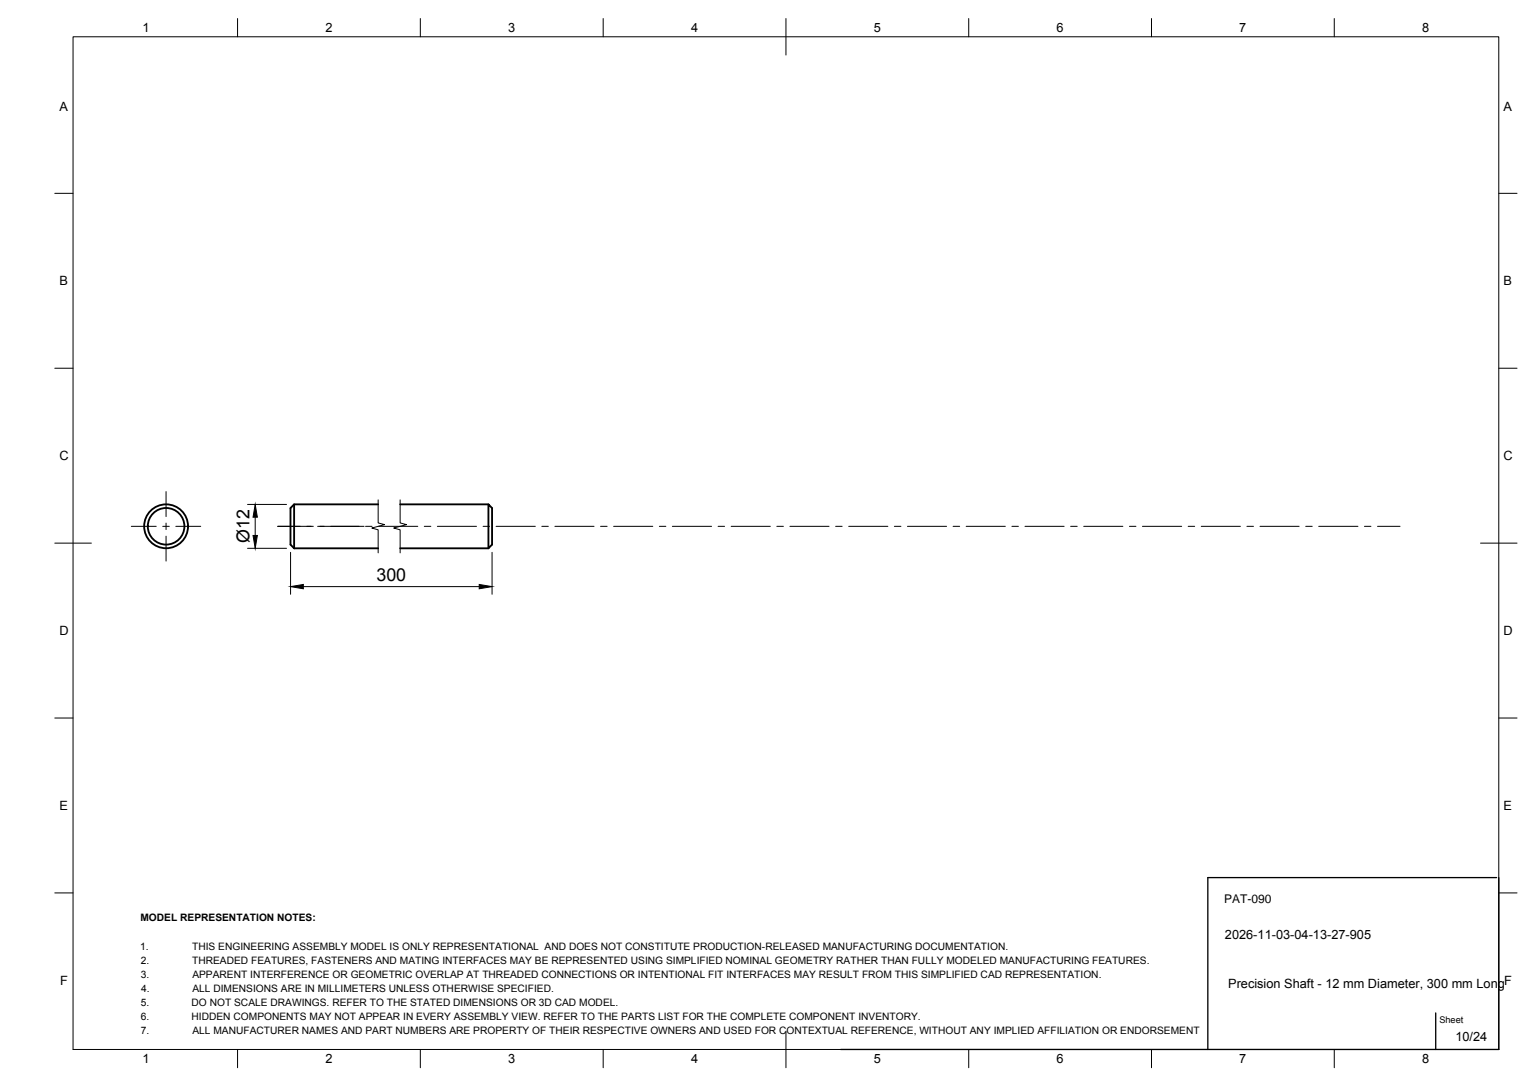
ISO-10303-21;
HEADER;
/* Generated by software containing ST-Developer
 * from STEP Tools, Inc. (www.steptools.com) 
 */

FILE_DESCRIPTION(
/* description */ ('Round-Shaft Linear Stage with Ball Bushings'),
/* implementation_level */ '2;1');

FILE_NAME(
/* name */ 'Precision Shaft - 12 mm Diameter, 300 mm Long.step',
/* time_stamp */ '2026-10-27T10:47:55-07:00',
/* author */ (''),
/* organization */ (''),
/* preprocessor_version */ 'ST-DEVELOPER v20.2',
/* originating_system */ 'Autodesk Translation Framework v15.17.0.0',
/* authorisation */ '');

FILE_SCHEMA (('AUTOMOTIVE_DESIGN { 1 0 10303 214 3 1 1 }'));
ENDSEC;

DATA;
#10=MECHANICAL_DESIGN_GEOMETRIC_PRESENTATION_REPRESENTATION('',(#307),#7835);
#243=CONICAL_SURFACE('',#4751,0.55,0.785398163397448);
#244=CONICAL_SURFACE('',#4757,0.55,0.785398163397441);
#265=SHAPE_REPRESENTATION_RELATIONSHIP('SRR','None',#7953,#286);
#286=ADVANCED_BREP_SHAPE_REPRESENTATION('',(#328),#7817);
#307=STYLED_ITEM('',(#8144),#328);
#328=MANIFOLD_SOLID_BREP('Body1',#4397);
#493=PLANE('',#4756);
#494=PLANE('',#4759);
#670=FACE_OUTER_BOUND('',#963,.T.);
#671=FACE_OUTER_BOUND('',#964,.T.);
#672=FACE_OUTER_BOUND('',#965,.T.);
#673=FACE_OUTER_BOUND('',#966,.T.);
#674=FACE_OUTER_BOUND('',#967,.T.);
#963=EDGE_LOOP('',(#3234,#3235,#3236,#3237));
#964=EDGE_LOOP('',(#3238,#3239,#3240,#3241));
#965=EDGE_LOOP('',(#3242));
#966=EDGE_LOOP('',(#3243,#3244,#3245,#3246));
#967=EDGE_LOOP('',(#3247));
#1329=LINE('',#6836,#1669);
#1330=LINE('',#6841,#1670);
#1331=LINE('',#6846,#1671);
#1669=VECTOR('',#5464,0.55);
#1670=VECTOR('',#5471,0.6);
#1671=VECTOR('',#5478,0.55);
#1969=CIRCLE('',#4752,0.6);
#1970=CIRCLE('',#4753,0.5);
#1971=CIRCLE('',#4755,0.6);
#1972=CIRCLE('',#4758,0.5);
#2198=VERTEX_POINT('',#6833);
#2199=VERTEX_POINT('',#6835);
#2200=VERTEX_POINT('',#6839);
#2201=VERTEX_POINT('',#6844);
#2585=EDGE_CURVE('',#2198,#2198,#1969,.T.);
#2586=EDGE_CURVE('',#2198,#2199,#1329,.T.);
#2587=EDGE_CURVE('',#2199,#2199,#1970,.T.);
#2588=EDGE_CURVE('',#2200,#2200,#1971,.T.);
#2589=EDGE_CURVE('',#2200,#2198,#1330,.T.);
#2590=EDGE_CURVE('',#2201,#2201,#1972,.T.);
#2591=EDGE_CURVE('',#2201,#2200,#1331,.T.);
#3234=ORIENTED_EDGE('',*,*,#2585,.T.);
#3235=ORIENTED_EDGE('',*,*,#2586,.T.);
#3236=ORIENTED_EDGE('',*,*,#2587,.T.);
#3237=ORIENTED_EDGE('',*,*,#2586,.F.);
#3238=ORIENTED_EDGE('',*,*,#2588,.F.);
#3239=ORIENTED_EDGE('',*,*,#2589,.T.);
#3240=ORIENTED_EDGE('',*,*,#2585,.F.);
#3241=ORIENTED_EDGE('',*,*,#2589,.F.);
#3242=ORIENTED_EDGE('',*,*,#2587,.F.);
#3243=ORIENTED_EDGE('',*,*,#2590,.T.);
#3244=ORIENTED_EDGE('',*,*,#2591,.T.);
#3245=ORIENTED_EDGE('',*,*,#2588,.T.);
#3246=ORIENTED_EDGE('',*,*,#2591,.F.);
#3247=ORIENTED_EDGE('',*,*,#2590,.F.);
#4072=CYLINDRICAL_SURFACE('',#4754,0.6);
#4189=ADVANCED_FACE('',(#670),#243,.T.);
#4190=ADVANCED_FACE('',(#671),#4072,.T.);
#4191=ADVANCED_FACE('',(#672),#493,.F.);
#4192=ADVANCED_FACE('',(#673),#244,.T.);
#4193=ADVANCED_FACE('',(#674),#494,.T.);
#4397=CLOSED_SHELL('',(#4189,#4190,#4191,#4192,#4193));
#4750=AXIS2_PLACEMENT_3D('',#6831,#5458,#5459);
#4751=AXIS2_PLACEMENT_3D('',#6832,#5460,#5461);
#4752=AXIS2_PLACEMENT_3D('',#6834,#5462,#5463);
#4753=AXIS2_PLACEMENT_3D('',#6837,#5465,#5466);
#4754=AXIS2_PLACEMENT_3D('',#6838,#5467,#5468);
#4755=AXIS2_PLACEMENT_3D('',#6840,#5469,#5470);
#4756=AXIS2_PLACEMENT_3D('',#6842,#5472,#5473);
#4757=AXIS2_PLACEMENT_3D('',#6843,#5474,#5475);
#4758=AXIS2_PLACEMENT_3D('',#6845,#5476,#5477);
#4759=AXIS2_PLACEMENT_3D('',#6847,#5479,#5480);
#5458=DIRECTION('axis',(0.,0.,1.));
#5459=DIRECTION('refdir',(1.,0.,0.));
#5460=DIRECTION('center_axis',(1.,0.,0.));
#5461=DIRECTION('ref_axis',(0.,0.,-1.));
#5462=DIRECTION('center_axis',(-1.,0.,0.));
#5463=DIRECTION('ref_axis',(0.,0.,-1.));
#5464=DIRECTION('',(-0.707106781186548,8.65956056235493E-17,-0.707106781186547));
#5465=DIRECTION('center_axis',(1.,0.,0.));
#5466=DIRECTION('ref_axis',(0.,0.,-1.));
#5467=DIRECTION('center_axis',(1.,0.,0.));
#5468=DIRECTION('ref_axis',(0.,0.,-1.));
#5469=DIRECTION('center_axis',(1.,0.,0.));
#5470=DIRECTION('ref_axis',(0.,0.,-1.));
#5471=DIRECTION('',(-1.,0.,0.));
#5472=DIRECTION('center_axis',(1.,0.,0.));
#5473=DIRECTION('ref_axis',(0.,0.,-1.));
#5474=DIRECTION('center_axis',(-1.,0.,0.));
#5475=DIRECTION('ref_axis',(0.,0.,-1.));
#5476=DIRECTION('center_axis',(-1.,0.,0.));
#5477=DIRECTION('ref_axis',(0.,0.,-1.));
#5478=DIRECTION('',(-0.707106781186553,-8.65956056235487E-17,0.707106781186542));
#5479=DIRECTION('center_axis',(1.,0.,0.));
#5480=DIRECTION('ref_axis',(0.,0.,-1.));
#6831=CARTESIAN_POINT('',(0.,0.,0.));
#6832=CARTESIAN_POINT('Origin',(0.05,0.,0.));
#6833=CARTESIAN_POINT('',(0.1,7.34788079488412E-17,0.6));
#6834=CARTESIAN_POINT('Origin',(0.1,0.,0.));
#6835=CARTESIAN_POINT('',(0.,-6.12323399573677E-17,0.5));
#6836=CARTESIAN_POINT('',(0.05,-6.73555739531044E-17,0.55));
#6837=CARTESIAN_POINT('Origin',(0.,0.,0.));
#6838=CARTESIAN_POINT('Origin',(0.,0.,0.));
#6839=CARTESIAN_POINT('',(29.9,-7.34788079488412E-17,0.6));
#6840=CARTESIAN_POINT('Origin',(29.9,0.,0.));
#6841=CARTESIAN_POINT('',(0.,-7.34788079488412E-17,0.6));
#6842=CARTESIAN_POINT('Origin',(0.,0.,0.));
#6843=CARTESIAN_POINT('Origin',(29.95,0.,0.));
#6844=CARTESIAN_POINT('',(30.,6.12323399573677E-17,0.5));
#6845=CARTESIAN_POINT('Origin',(30.,0.,0.));
#6846=CARTESIAN_POINT('',(29.95,-6.73555739531044E-17,0.55));
#6847=CARTESIAN_POINT('Origin',(30.,0.,0.));
#7791=UNCERTAINTY_MEASURE_WITH_UNIT(LENGTH_MEASURE(0.001),#7836,
'DISTANCE_ACCURACY_VALUE',
'Maximum model space distance between geometric entities at asserted c
onnectivities');
#7809=UNCERTAINTY_MEASURE_WITH_UNIT(LENGTH_MEASURE(0.001),#7836,
'DISTANCE_ACCURACY_VALUE',
'Maximum model space distance between geometric entities at asserted c
onnectivities');
#7817=(
GEOMETRIC_REPRESENTATION_CONTEXT(3)
GLOBAL_UNCERTAINTY_ASSIGNED_CONTEXT((#7791))
GLOBAL_UNIT_ASSIGNED_CONTEXT((#7836,#7838,#7839))
REPRESENTATION_CONTEXT('','3D')
);
#7835=(
GEOMETRIC_REPRESENTATION_CONTEXT(3)
GLOBAL_UNCERTAINTY_ASSIGNED_CONTEXT((#7809))
GLOBAL_UNIT_ASSIGNED_CONTEXT((#7836,#7838,#7839))
REPRESENTATION_CONTEXT('','3D')
);
#7836=(
LENGTH_UNIT()
NAMED_UNIT(*)
SI_UNIT(.CENTI.,.METRE.)
);
#7838=(
NAMED_UNIT(*)
PLANE_ANGLE_UNIT()
SI_UNIT($,.RADIAN.)
);
#7839=(
NAMED_UNIT(*)
SI_UNIT($,.STERADIAN.)
SOLID_ANGLE_UNIT()
);
#7847=SHAPE_DEFINITION_REPRESENTATION(#7872,#7953);
#7872=PRODUCT_DEFINITION_SHAPE('',$,#7979);
#7953=SHAPE_REPRESENTATION('',(#4750),#7817);
#7971=PRODUCT_DEFINITION_CONTEXT('part definition',#8048,'design');
#7979=PRODUCT_DEFINITION(
'Precision Shaft - 12 mm Diameter, 300 mm Long',
'Precision Shaft - 12 mm Diameter, 300 mm Long',#8004,#7971);
#8004=PRODUCT_DEFINITION_FORMATION('',$,#8057);
#8048=APPLICATION_CONTEXT(
'Core Data for Automotive Mechanical Design Process');
#8049=PRODUCT_CONTEXT('part definition',#8048,'mechanical');
#8057=PRODUCT('Precision Shaft - 12 mm Diameter, 300 mm Long',
'Precision Shaft - 12 mm Diameter, 300 mm Long',
'Precision Shaft - 12 mm Diameter, 300 mm Long',(#8049));
#8138=COLOUR_RGB('Grey',0.48,0.52,0.57);
#8139=FILL_AREA_STYLE_COLOUR('',#8138);
#8140=FILL_AREA_STYLE('',(#8139));
#8141=SURFACE_STYLE_FILL_AREA(#8140);
#8142=SURFACE_SIDE_STYLE('',(#8141));
#8143=SURFACE_STYLE_USAGE(.BOTH.,#8142);
#8144=PRESENTATION_STYLE_ASSIGNMENT((#8143));
ENDSEC;
END-ISO-10303-21;
